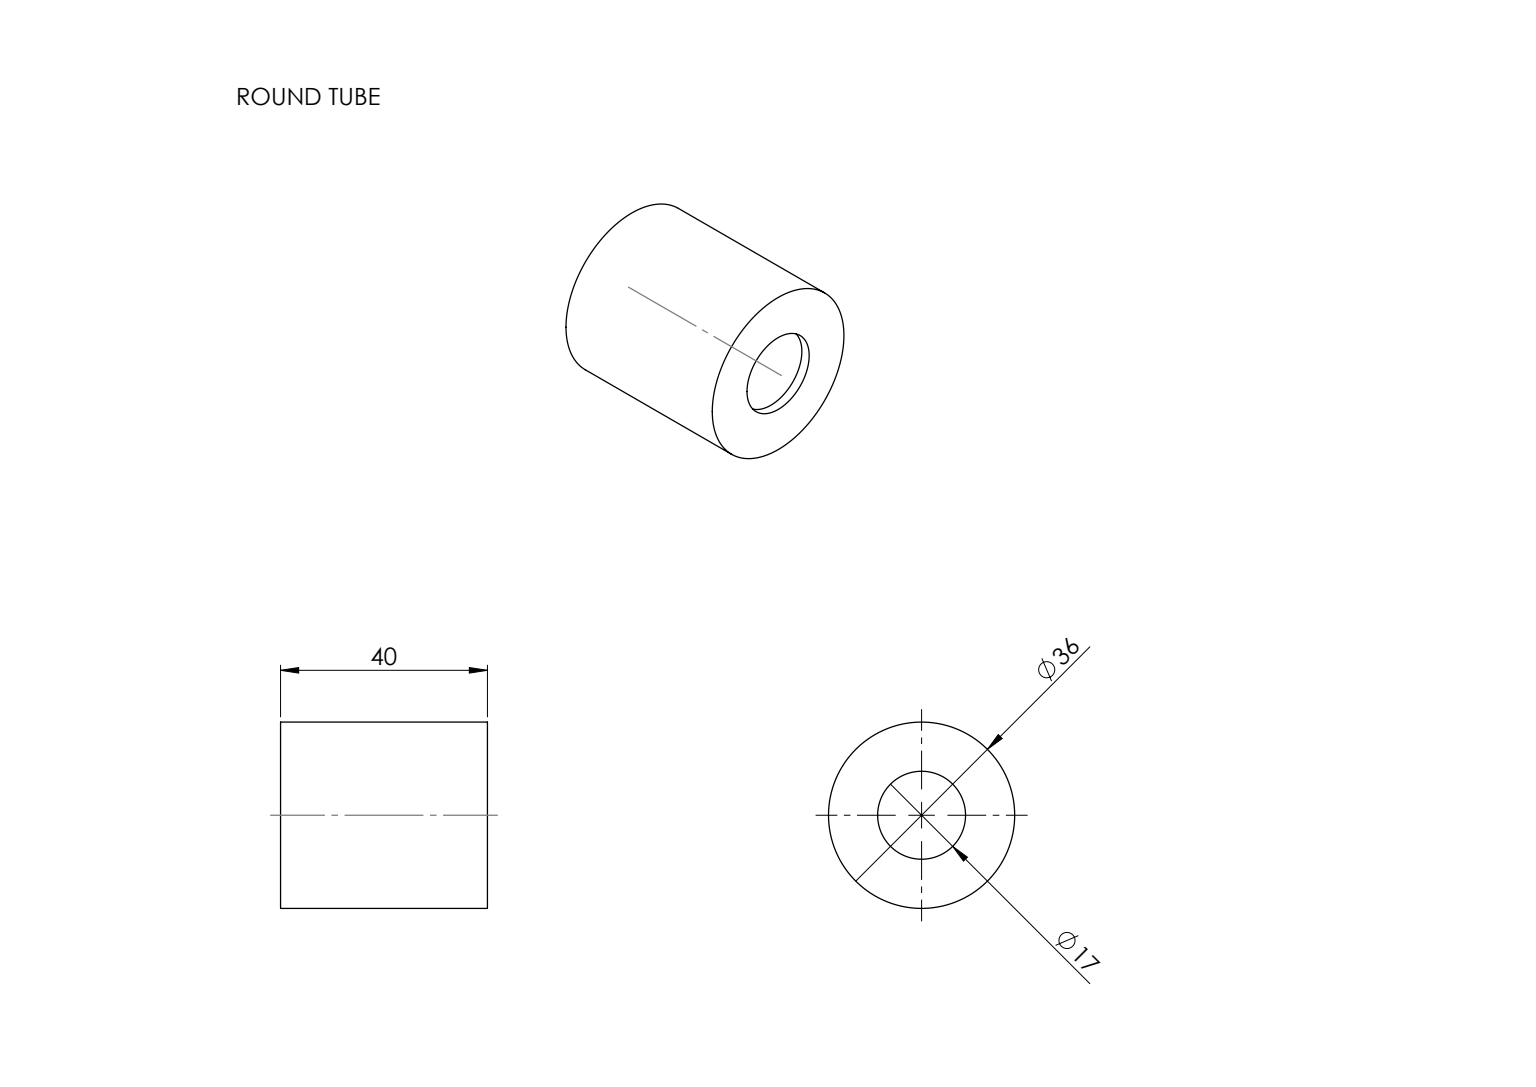
ISO-10303-21;
HEADER;
FILE_DESCRIPTION (('STEP AP214'),
    '1' );
FILE_NAME ('round tube.step',
    '2026-10-08T13:22:57',
    ( '' ),
    ( '' ),
    'SwSTEP 2.0',
    'SolidWorks 2026',
    '' );
FILE_SCHEMA (( 'AUTOMOTIVE_DESIGN' ));
ENDSEC;

DATA;
#17=DIRECTION ( 'NONE',  ( 0.000000000000000000, 0.000000000000000000, 1.000000000000000000 ) ) ;
#49=DIRECTION ( 'NONE',  ( -1.000000000000000000, 0.000000000000000000, -0.000000000000000000 ) ) ;
#62=CARTESIAN_POINT ( 'NONE',  ( -108.0000000000000284, 0.000000000000000000, 18.00000000000000000 ) ) ;
#71=FACE_OUTER_BOUND ( 'NONE', #2223, .T. ) ;
#103=EDGE_LOOP ( 'NONE', ( #4875, #2005 ) ) ;
#211=ADVANCED_FACE ( 'NONE', ( #9553 ), #5041, .F. ) ;
#245=CARTESIAN_POINT ( 'NONE',  ( 0.000000000000000000, 0.000000000000000000, 0.000000000000000000 ) ) ;
#254=MANIFOLD_SOLID_BREP ( 'Revolve-Thin1', #5480 ) ;
#268=EDGE_CURVE ( 'NONE', #3156, #7778, #4308, .T. ) ;
#280=FACE_OUTER_BOUND ( 'NONE', #4887, .T. ) ;
#290=EDGE_CURVE ( 'NONE', #9194, #8643, #8941, .T. ) ;
#357=( GEOMETRIC_REPRESENTATION_CONTEXT ( 3 ) GLOBAL_UNCERTAINTY_ASSIGNED_CONTEXT ( ( #1022 ) ) GLOBAL_UNIT_ASSIGNED_CONTEXT ( ( #599, #1315, #9183 ) ) REPRESENTATION_CONTEXT ( 'NONE', 'WORKASPACE' ) );
#358=( GEOMETRIC_REPRESENTATION_CONTEXT ( 3 ) GLOBAL_UNCERTAINTY_ASSIGNED_CONTEXT ( ( #7416 ) ) GLOBAL_UNIT_ASSIGNED_CONTEXT ( ( #3591, #997, #9684 ) ) REPRESENTATION_CONTEXT ( 'NONE', 'WORKASPACE' ) );
#438=EDGE_LOOP ( 'NONE', ( #4414, #892, #4751, #3837 ) ) ;
#465=ORIENTED_EDGE ( 'NONE', *, *, #2286, .F. ) ;
#494=PRODUCT_DEFINITION_CONTEXT ( 'detailed design', #8367, 'design' ) ;
#512=PRODUCT_CONTEXT ( 'NONE', #7716, 'mechanical' ) ;
#515=ORIENTED_EDGE ( 'NONE', *, *, #5831, .F. ) ;
#561=ADVANCED_FACE ( 'NONE', ( #71, #5593 ), #1530, .F. ) ;
#599=( LENGTH_UNIT ( ) NAMED_UNIT ( * ) SI_UNIT ( .MILLI., .METRE. ) );
#605=FILL_AREA_STYLE ('',( #8456 ) ) ;
#729=CARTESIAN_POINT ( 'NONE',  ( -108.0000000000000284, 2.204364238465235822E-15, -18.00000000000000355 ) ) ;
#740=EDGE_CURVE ( 'NONE', #7778, #3156, #4627, .T. ) ;
#763=DIRECTION ( 'NONE',  ( 0.000000000000000000, 0.000000000000000000, 1.000000000000000000 ) ) ;
#826=AXIS2_PLACEMENT_3D ( 'NONE', #1580, #4054, #7874 ) ;
#832=AXIS2_PLACEMENT_3D ( 'NONE', #8024, #7249, #6413 ) ;
#851=COLOUR_RGB ( '', 0.40784314, 0.44705882, 0.49803922) ;
#892=ORIENTED_EDGE ( 'NONE', *, *, #7551, .T. ) ;
#909=DIRECTION ( 'NONE',  ( -1.000000000000000000, -0.000000000000000000, -0.000000000000000000 ) ) ;
#932=ADVANCED_FACE ( 'NONE', ( #8639, #3149 ), #7183, .T. ) ;
#997=( NAMED_UNIT ( * ) PLANE_ANGLE_UNIT ( ) SI_UNIT ( $, .RADIAN. ) );
#1022=UNCERTAINTY_MEASURE_WITH_UNIT (LENGTH_MEASURE( 1.000000000000000082E-05 ), #599, 'distance_accuracy_value', 'NONE');
#1046=CIRCLE ( 'NONE', #1889, 15.99999999999999645 ) ;
#1072=CARTESIAN_POINT ( 'NONE',  ( -108.0000000000000284, 0.000000000000000000, 0.000000000000000000 ) ) ;
#1082=CYLINDRICAL_SURFACE ( 'NONE', #9749, 18.00000000000000355 ) ;
#1084=ORIENTED_EDGE ( 'NONE', *, *, #1371, .T. ) ;
#1137=ORIENTED_EDGE ( 'NONE', *, *, #2286, .T. ) ;
#1152=CARTESIAN_POINT ( 'NONE',  ( -108.0000000000000284, 0.000000000000000000, 0.000000000000000000 ) ) ;
#1175=ADVANCED_FACE ( 'NONE', ( #2510 ), #3234, .T. ) ;
#1211=LINE ( 'NONE', #6933, #2321 ) ;
#1315=( NAMED_UNIT ( * ) PLANE_ANGLE_UNIT ( ) SI_UNIT ( $, .RADIAN. ) );
#1371=EDGE_CURVE ( 'NONE', #3156, #3923, #3906, .T. ) ;
#1433=( LENGTH_UNIT ( ) NAMED_UNIT ( * ) SI_UNIT ( .MILLI., .METRE. ) );
#1457=CARTESIAN_POINT ( 'NONE',  ( -108.0000000000000284, 15.99999999999999645, 0.000000000000000000 ) ) ;
#1476=ADVANCED_FACE ( 'NONE', ( #9765 ), #1082, .T. ) ;
#1500=CARTESIAN_POINT ( 'NONE',  ( -108.0000000000000284, 0.000000000000000000, 15.99999999999999645 ) ) ;
#1517=COLOUR_RGB ( '', 0.40784314, 0.44705882, 0.49803922) ;
#1529=DIRECTION ( 'NONE',  ( -1.000000000000000000, 0.000000000000000000, -0.000000000000000000 ) ) ;
#1530=PLANE ( 'NONE',  #826 ) ;
#1577=CARTESIAN_POINT ( 'NONE',  ( -70.00000000000001421, 0.000000000000000000, 0.000000000000000000 ) ) ;
#1580=CARTESIAN_POINT ( 'NONE',  ( -68.00000000000001421, 8.500000000000000000, 0.000000000000000000 ) ) ;
#1624=CARTESIAN_POINT ( 'NONE',  ( -108.0000000000000284, 0.000000000000000000, 0.000000000000000000 ) ) ;
#1627=DIRECTION ( 'NONE',  ( -0.000000000000000000, 0.000000000000000000, 1.000000000000000000 ) ) ;
#1642=UNCERTAINTY_MEASURE_WITH_UNIT (LENGTH_MEASURE( 1.000000000000000082E-05 ), #1433, 'distance_accuracy_value', 'NONE');
#1673=DIRECTION ( 'NONE',  ( -1.000000000000000000, -0.000000000000000000, -0.000000000000000000 ) ) ;
#1678=CARTESIAN_POINT ( 'NONE',  ( -70.00000000000001421, 0.000000000000000000, 16.00000000000000000 ) ) ;
#1695=CARTESIAN_POINT ( 'NONE',  ( -108.0000000000000284, 0.000000000000000000, 0.000000000000000000 ) ) ;
#1829=CYLINDRICAL_SURFACE ( 'NONE', #3463, 16.00000000000000000 ) ;
#1832=AXIS2_PLACEMENT_3D ( 'NONE', #1072, #7466, #8187 ) ;
#1874=PRODUCT ( 'round tube', 'round tube', '', ( #512 ) ) ;
#1889=AXIS2_PLACEMENT_3D ( 'NONE', #1152, #1926, #9840 ) ;
#1926=DIRECTION ( 'NONE',  ( -1.000000000000000000, -0.000000000000000000, -0.000000000000000000 ) ) ;
#1927=CIRCLE ( 'NONE', #8535, 8.500000000000000000 ) ;
#1974=DIRECTION ( 'NONE',  ( 0.000000000000000000, 0.000000000000000000, 1.000000000000000000 ) ) ;
#2003=VERTEX_POINT ( 'NONE', #3029 ) ;
#2005=ORIENTED_EDGE ( 'NONE', *, *, #5772, .T. ) ;
#2018=CARTESIAN_POINT ( 'NONE',  ( -108.0000000000000284, 2.204364238465235428E-15, -18.00000000000000000 ) ) ;
#2037=PRODUCT_DEFINITION_SHAPE ( 'NONE', 'NONE',  #4346 ) ;
#2045=( NAMED_UNIT ( * ) SI_UNIT ( $, .STERADIAN. ) SOLID_ANGLE_UNIT ( ) );
#2095=AXIS2_PLACEMENT_3D ( 'NONE', #4772, #6463, #6557 ) ;
#2131=DIRECTION ( 'NONE',  ( -1.000000000000000000, -0.000000000000000000, -0.000000000000000000 ) ) ;
#2223=EDGE_LOOP ( 'NONE', ( #7638, #5766 ) ) ;
#2224=LINE ( 'NONE', #729, #9042 ) ;
#2228=EDGE_CURVE ( 'NONE', #6421, #9282, #4166, .T. ) ;
#2243=ORIENTED_EDGE ( 'NONE', *, *, #5831, .T. ) ;
#2252=DIRECTION ( 'NONE',  ( 0.000000000000000000, 0.000000000000000000, 1.000000000000000000 ) ) ;
#2286=EDGE_CURVE ( 'NONE', #9360, #3923, #3473, .T. ) ;
#2321=VECTOR ( 'NONE', #8550, 1000.000000000000000 ) ;
#2344=ORIENTED_EDGE ( 'NONE', *, *, #3789, .T. ) ;
#2413=ADVANCED_BREP_SHAPE_REPRESENTATION ( '', ( #254, #3995 ), #6945 ) ;
#2510=FACE_OUTER_BOUND ( 'NONE', #6282, .T. ) ;
#2527=VECTOR ( 'NONE', #6510, 1000.000000000000000 ) ;
#2554=CARTESIAN_POINT ( 'NONE',  ( -108.0000000000000284, 0.000000000000000000, 0.000000000000000000 ) ) ;
#2576=EDGE_LOOP ( 'NONE', ( #7299, #6905, #10175, #9434 ) ) ;
#2657=CARTESIAN_POINT ( 'NONE',  ( -108.0000000000000284, 0.000000000000000000, 0.000000000000000000 ) ) ;
#2669=DIRECTION ( 'NONE',  ( 0.000000000000000000, 0.000000000000000000, 1.000000000000000000 ) ) ;
#2678=ORIENTED_EDGE ( 'NONE', *, *, #5440, .F. ) ;
#2699=EDGE_CURVE ( 'NONE', #5232, #8643, #1211, .T. ) ;
#2721=ORIENTED_EDGE ( 'NONE', *, *, #8828, .F. ) ;
#2805=CIRCLE ( 'NONE', #8595, 18.00000000000000000 ) ;
#2816=CIRCLE ( 'NONE', #4642, 18.00000000000000355 ) ;
#2882=ORIENTED_EDGE ( 'NONE', *, *, #5772, .F. ) ;
#2885=ADVANCED_FACE ( 'NONE', ( #7092 ), #7730, .F. ) ;
#2988=AXIS2_PLACEMENT_3D ( 'NONE', #4365, #5955, #6053 ) ;
#3026=SURFACE_STYLE_USAGE ( .BOTH. , #3753 ) ;
#3029=CARTESIAN_POINT ( 'NONE',  ( -68.00000000000001421, 2.204364238465235822E-15, -18.00000000000000355 ) ) ;
#3066=EDGE_CURVE ( 'NONE', #6680, #9282, #1927, .T. ) ;
#3072=CARTESIAN_POINT ( 'NONE',  ( -68.00000000000001421, 0.000000000000000000, 0.000000000000000000 ) ) ;
#3149=FACE_BOUND ( 'NONE', #4435, .T. ) ;
#3156=VERTEX_POINT ( 'NONE', #1678 ) ;
#3186=AXIS2_PLACEMENT_3D ( 'NONE', #8225, #2131, #1974 ) ;
#3234=CYLINDRICAL_SURFACE ( 'NONE', #7095, 18.00000000000000355 ) ;
#3245=CARTESIAN_POINT ( 'NONE',  ( -108.0000000000000284, 0.000000000000000000, 0.000000000000000000 ) ) ;
#3271=CARTESIAN_POINT ( 'NONE',  ( -68.00000000000001421, 0.000000000000000000, 18.00000000000000355 ) ) ;
#3292=EDGE_CURVE ( 'NONE', #9282, #6680, #10186, .T. ) ;
#3294=DIRECTION ( 'NONE',  ( -1.000000000000000000, -0.000000000000000000, -0.000000000000000000 ) ) ;
#3339=DIRECTION ( 'NONE',  ( -1.000000000000000000, -0.000000000000000000, -0.000000000000000000 ) ) ;
#3453=STYLED_ITEM ( 'NONE', ( #5194 ), #254 ) ;
#3462=VECTOR ( 'NONE', #8822, 1000.000000000000000 ) ;
#3463=AXIS2_PLACEMENT_3D ( 'NONE', #2554, #909, #7928 ) ;
#3473=CIRCLE ( 'NONE', #9920, 15.99999999999999645 ) ;
#3502=EDGE_LOOP ( 'NONE', ( #9090, #6134 ) ) ;
#3591=( LENGTH_UNIT ( ) NAMED_UNIT ( * ) SI_UNIT ( .MILLI., .METRE. ) );
#3650=ORIENTED_EDGE ( 'NONE', *, *, #8828, .T. ) ;
#3753=SURFACE_SIDE_STYLE ('',( #6946 ) ) ;
#3789=EDGE_CURVE ( 'NONE', #2003, #9194, #2224, .T. ) ;
#3800=FACE_BOUND ( 'NONE', #10074, .T. ) ;
#3837=ORIENTED_EDGE ( 'NONE', *, *, #290, .F. ) ;
#3901=PLANE ( 'NONE',  #10093 ) ;
#3906=LINE ( 'NONE', #4060, #3462 ) ;
#3923=VERTEX_POINT ( 'NONE', #1500 ) ;
#3995=AXIS2_PLACEMENT_3D ( 'NONE', #245, #8930, #7419 ) ;
#4054=DIRECTION ( 'NONE',  ( -1.000000000000000000, 0.000000000000000000, -0.000000000000000000 ) ) ;
#4060=CARTESIAN_POINT ( 'NONE',  ( -108.0000000000000284, 0.000000000000000000, 16.00000000000000000 ) ) ;
#4104=CARTESIAN_POINT ( 'NONE',  ( -108.0000000000000284, 0.000000000000000000, 8.500000000000000000 ) ) ;
#4114=CARTESIAN_POINT ( 'NONE',  ( -108.0000000000000284, 1.040949779275250140E-15, -8.500000000000000000 ) ) ;
#4137=AXIS2_PLACEMENT_3D ( 'NONE', #3072, #6216, #8452 ) ;
#4166=LINE ( 'NONE', #4114, #4962 ) ;
#4168=DIRECTION ( 'NONE',  ( 0.000000000000000000, 0.000000000000000000, 1.000000000000000000 ) ) ;
#4201=LINE ( 'NONE', #4104, #2527 ) ;
#4259=ORIENTED_EDGE ( 'NONE', *, *, #290, .T. ) ;
#4308=CIRCLE ( 'NONE', #7941, 16.00000000000000000 ) ;
#4346=PRODUCT_DEFINITION ( 'UNKNOWN', '', #9394, #494 ) ;
#4352=AXIS2_PLACEMENT_3D ( 'NONE', #6148, #7768, #7815 ) ;
#4365=CARTESIAN_POINT ( 'NONE',  ( -108.0000000000000284, 0.000000000000000000, 0.000000000000000000 ) ) ;
#4414=ORIENTED_EDGE ( 'NONE', *, *, #3789, .F. ) ;
#4435=EDGE_LOOP ( 'NONE', ( #515, #465 ) ) ;
#4461=ORIENTED_EDGE ( 'NONE', *, *, #2699, .F. ) ;
#4464=AXIS2_PLACEMENT_3D ( 'NONE', #4630, #6262, #2252 ) ;
#4467=VECTOR ( 'NONE', #1673, 1000.000000000000000 ) ;
#4485=ORIENTED_EDGE ( 'NONE', *, *, #3292, .T. ) ;
#4526=FILL_AREA_STYLE_COLOUR ( '', #851 ) ;
#4534=CIRCLE ( 'NONE', #4352, 8.500000000000000000 ) ;
#4550=SHAPE_REPRESENTATION ( 'round tube', ( #3995 ), #6945 ) ;
#4575=DIRECTION ( 'NONE',  ( 0.000000000000000000, 0.000000000000000000, 1.000000000000000000 ) ) ;
#4627=CIRCLE ( 'NONE', #832, 16.00000000000000000 ) ;
#4630=CARTESIAN_POINT ( 'NONE',  ( -108.0000000000000284, 0.000000000000000000, 0.000000000000000000 ) ) ;
#4642=AXIS2_PLACEMENT_3D ( 'NONE', #5903, #9135, #4168 ) ;
#4648=AXIS2_PLACEMENT_3D ( 'NONE', #1624, #4675, #17 ) ;
#4675=DIRECTION ( 'NONE',  ( -1.000000000000000000, -0.000000000000000000, -0.000000000000000000 ) ) ;
#4751=ORIENTED_EDGE ( 'NONE', *, *, #2699, .T. ) ;
#4772=CARTESIAN_POINT ( 'NONE',  ( -70.00000000000001421, 0.000000000000000000, 0.000000000000000000 ) ) ;
#4875=ORIENTED_EDGE ( 'NONE', *, *, #6005, .T. ) ;
#4887=EDGE_LOOP ( 'NONE', ( #8548, #9088, #1137, #10177 ) ) ;
#4962=VECTOR ( 'NONE', #3339, 1000.000000000000000 ) ;
#5041=CYLINDRICAL_SURFACE ( 'NONE', #1832, 8.500000000000000000 ) ;
#5130=CIRCLE ( 'NONE', #4137, 18.00000000000000355 ) ;
#5154=ADVANCED_FACE ( 'NONE', ( #5546, #3800 ), #3901, .T. ) ;
#5194=PRESENTATION_STYLE_ASSIGNMENT (( #7683 ) ) ;
#5232=VERTEX_POINT ( 'NONE', #3271 ) ;
#5237=DIRECTION ( 'NONE',  ( -1.000000000000000000, -0.000000000000000000, -0.000000000000000000 ) ) ;
#5440=EDGE_CURVE ( 'NONE', #10061, #6680, #4201, .T. ) ;
#5445=CARTESIAN_POINT ( 'NONE',  ( -70.00000000000001421, 8.500000000000000000, 0.000000000000000000 ) ) ;
#5449=CARTESIAN_POINT ( 'NONE',  ( -70.00000000000001421, 1.959434878635765131E-15, -16.00000000000000000 ) ) ;
#5480=CLOSED_SHELL ( 'NONE', ( #8027, #211, #1175, #1476, #561, #2885, #5154, #7882, #932 ) ) ;
#5546=FACE_OUTER_BOUND ( 'NONE', #3502, .T. ) ;
#5593=FACE_BOUND ( 'NONE', #103, .T. ) ;
#5683=CARTESIAN_POINT ( 'NONE',  ( -68.00000000000001421, 1.040949779275250140E-15, -8.500000000000000000 ) ) ;
#5766=ORIENTED_EDGE ( 'NONE', *, *, #7551, .F. ) ;
#5772=EDGE_CURVE ( 'NONE', #6421, #10061, #7971, .T. ) ;
#5831=EDGE_CURVE ( 'NONE', #3923, #9360, #1046, .T. ) ;
#5903=CARTESIAN_POINT ( 'NONE',  ( -68.00000000000001421, 0.000000000000000000, 0.000000000000000000 ) ) ;
#5955=DIRECTION ( 'NONE',  ( -1.000000000000000000, -0.000000000000000000, -0.000000000000000000 ) ) ;
#6005=EDGE_CURVE ( 'NONE', #10061, #6421, #4534, .T. ) ;
#6053=DIRECTION ( 'NONE',  ( 0.000000000000000000, 0.000000000000000000, 1.000000000000000000 ) ) ;
#6134=ORIENTED_EDGE ( 'NONE', *, *, #740, .T. ) ;
#6148=CARTESIAN_POINT ( 'NONE',  ( -68.00000000000001421, 0.000000000000000000, 0.000000000000000000 ) ) ;
#6158=DIRECTION ( 'NONE',  ( -1.000000000000000000, -0.000000000000000000, -0.000000000000000000 ) ) ;
#6168=PRESENTATION_STYLE_ASSIGNMENT (( #3026 ) ) ;
#6216=DIRECTION ( 'NONE',  ( -1.000000000000000000, -0.000000000000000000, -0.000000000000000000 ) ) ;
#6262=DIRECTION ( 'NONE',  ( -1.000000000000000000, -0.000000000000000000, -0.000000000000000000 ) ) ;
#6282=EDGE_LOOP ( 'NONE', ( #7580, #2344, #2721, #4461 ) ) ;
#6355=CARTESIAN_POINT ( 'NONE',  ( -108.0000000000000284, 1.959434878635765131E-15, -16.00000000000000000 ) ) ;
#6413=DIRECTION ( 'NONE',  ( 0.000000000000000000, 0.000000000000000000, 1.000000000000000000 ) ) ;
#6421=VERTEX_POINT ( 'NONE', #5683 ) ;
#6463=DIRECTION ( 'NONE',  ( -1.000000000000000000, -0.000000000000000000, -0.000000000000000000 ) ) ;
#6510=DIRECTION ( 'NONE',  ( -1.000000000000000000, -0.000000000000000000, -0.000000000000000000 ) ) ;
#6551=CARTESIAN_POINT ( 'NONE',  ( -70.00000000000001421, 1.040949779275250140E-15, -8.500000000000000000 ) ) ;
#6557=DIRECTION ( 'NONE',  ( 0.000000000000000000, 0.000000000000000000, 1.000000000000000000 ) ) ;
#6680=VERTEX_POINT ( 'NONE', #8366 ) ;
#6795=SHAPE_DEFINITION_REPRESENTATION ( #2037, #4550 ) ;
#6905=ORIENTED_EDGE ( 'NONE', *, *, #6005, .F. ) ;
#6933=CARTESIAN_POINT ( 'NONE',  ( -108.0000000000000284, 0.000000000000000000, 18.00000000000000355 ) ) ;
#6945=( GEOMETRIC_REPRESENTATION_CONTEXT ( 3 ) GLOBAL_UNCERTAINTY_ASSIGNED_CONTEXT ( ( #1642 ) ) GLOBAL_UNIT_ASSIGNED_CONTEXT ( ( #1433, #9343, #2045 ) ) REPRESENTATION_CONTEXT ( 'NONE', 'WORKASPACE' ) );
#6946=SURFACE_STYLE_FILL_AREA ( #605 ) ;
#7025=DIRECTION ( 'NONE',  ( -0.000000000000000000, 0.000000000000000000, 1.000000000000000000 ) ) ;
#7049=FACE_OUTER_BOUND ( 'NONE', #7278, .T. ) ;
#7075=CARTESIAN_POINT ( 'NONE',  ( -68.00000000000001421, 0.000000000000000000, 8.500000000000000000 ) ) ;
#7086=LINE ( 'NONE', #6355, #4467 ) ;
#7092=FACE_OUTER_BOUND ( 'NONE', #2576, .T. ) ;
#7095=AXIS2_PLACEMENT_3D ( 'NONE', #1695, #7213, #763 ) ;
#7144=DIRECTION ( 'NONE',  ( -1.000000000000000000, -0.000000000000000000, -0.000000000000000000 ) ) ;
#7179=EDGE_CURVE ( 'NONE', #5232, #2003, #2816, .T. ) ;
#7183=PLANE ( 'NONE',  #8415 ) ;
#7213=DIRECTION ( 'NONE',  ( -1.000000000000000000, -0.000000000000000000, -0.000000000000000000 ) ) ;
#7249=DIRECTION ( 'NONE',  ( -1.000000000000000000, -0.000000000000000000, -0.000000000000000000 ) ) ;
#7278=EDGE_LOOP ( 'NONE', ( #9525, #8525, #1084, #2243 ) ) ;
#7299=ORIENTED_EDGE ( 'NONE', *, *, #2228, .F. ) ;
#7347=SHAPE_REPRESENTATION_RELATIONSHIP ( 'NONE' , 'NONE' ,  #4550, #2413 ) ;
#7411=DIRECTION ( 'NONE',  ( 0.000000000000000000, 0.000000000000000000, 1.000000000000000000 ) ) ;
#7416=UNCERTAINTY_MEASURE_WITH_UNIT (LENGTH_MEASURE( 1.000000000000000082E-05 ), #3591, 'distance_accuracy_value', 'NONE');
#7419=DIRECTION ( 'NONE',  ( 1.000000000000000000, 0.000000000000000000, 0.000000000000000000 ) ) ;
#7445=MECHANICAL_DESIGN_GEOMETRIC_PRESENTATION_REPRESENTATION('',(#3453),#357);
#7466=DIRECTION ( 'NONE',  ( -1.000000000000000000, -0.000000000000000000, -0.000000000000000000 ) ) ;
#7518=SURFACE_STYLE_FILL_AREA ( #7625 ) ;
#7551=EDGE_CURVE ( 'NONE', #2003, #5232, #5130, .T. ) ;
#7580=ORIENTED_EDGE ( 'NONE', *, *, #7179, .T. ) ;
#7625=FILL_AREA_STYLE ('',( #4526 ) ) ;
#7638=ORIENTED_EDGE ( 'NONE', *, *, #7179, .F. ) ;
#7683=SURFACE_STYLE_USAGE ( .BOTH. , #9955 ) ;
#7716=APPLICATION_CONTEXT ( 'automotive_design' ) ;
#7730=CYLINDRICAL_SURFACE ( 'NONE', #4648, 8.500000000000000000 ) ;
#7753=EDGE_LOOP ( 'NONE', ( #2882, #7908, #4485, #2678 ) ) ;
#7768=DIRECTION ( 'NONE',  ( -1.000000000000000000, -0.000000000000000000, -0.000000000000000000 ) ) ;
#7778=VERTEX_POINT ( 'NONE', #5449 ) ;
#7792=STYLED_ITEM ( 'NONE', ( #6168 ), #2413 ) ;
#7815=DIRECTION ( 'NONE',  ( 0.000000000000000000, 0.000000000000000000, 1.000000000000000000 ) ) ;
#7874=DIRECTION ( 'NONE',  ( -0.000000000000000000, 0.000000000000000000, 1.000000000000000000 ) ) ;
#7882=ADVANCED_FACE ( 'NONE', ( #7049 ), #9342, .F. ) ;
#7908=ORIENTED_EDGE ( 'NONE', *, *, #2228, .T. ) ;
#7928=DIRECTION ( 'NONE',  ( 0.000000000000000000, 0.000000000000000000, 1.000000000000000000 ) ) ;
#7941=AXIS2_PLACEMENT_3D ( 'NONE', #8342, #5237, #9901 ) ;
#7971=CIRCLE ( 'NONE', #3186, 8.500000000000000000 ) ;
#8024=CARTESIAN_POINT ( 'NONE',  ( -70.00000000000001421, 0.000000000000000000, 0.000000000000000000 ) ) ;
#8027=ADVANCED_FACE ( 'NONE', ( #280 ), #1829, .F. ) ;
#8068=DIRECTION ( 'NONE',  ( 0.000000000000000000, 0.000000000000000000, 1.000000000000000000 ) ) ;
#8135=DIRECTION ( 'NONE',  ( -1.000000000000000000, -0.000000000000000000, -0.000000000000000000 ) ) ;
#8187=DIRECTION ( 'NONE',  ( 0.000000000000000000, 0.000000000000000000, 1.000000000000000000 ) ) ;
#8197=ORIENTED_EDGE ( 'NONE', *, *, #3066, .F. ) ;
#8225=CARTESIAN_POINT ( 'NONE',  ( -68.00000000000001421, 0.000000000000000000, 0.000000000000000000 ) ) ;
#8342=CARTESIAN_POINT ( 'NONE',  ( -70.00000000000001421, 0.000000000000000000, 0.000000000000000000 ) ) ;
#8366=CARTESIAN_POINT ( 'NONE',  ( -70.00000000000001421, 0.000000000000000000, 8.500000000000000000 ) ) ;
#8367=APPLICATION_CONTEXT ( 'automotive_design' ) ;
#8415=AXIS2_PLACEMENT_3D ( 'NONE', #1457, #49, #7025 ) ;
#8452=DIRECTION ( 'NONE',  ( 0.000000000000000000, 0.000000000000000000, 1.000000000000000000 ) ) ;
#8456=FILL_AREA_STYLE_COLOUR ( '', #1517 ) ;
#8525=ORIENTED_EDGE ( 'NONE', *, *, #268, .F. ) ;
#8535=AXIS2_PLACEMENT_3D ( 'NONE', #1577, #6158, #4575 ) ;
#8548=ORIENTED_EDGE ( 'NONE', *, *, #740, .F. ) ;
#8550=DIRECTION ( 'NONE',  ( -1.000000000000000000, -0.000000000000000000, -0.000000000000000000 ) ) ;
#8595=AXIS2_PLACEMENT_3D ( 'NONE', #9581, #7144, #8068 ) ;
#8614=MECHANICAL_DESIGN_GEOMETRIC_PRESENTATION_REPRESENTATION('',(#7792),#358);
#8639=FACE_OUTER_BOUND ( 'NONE', #9147, .T. ) ;
#8643=VERTEX_POINT ( 'NONE', #62 ) ;
#8822=DIRECTION ( 'NONE',  ( -1.000000000000000000, -0.000000000000000000, -0.000000000000000000 ) ) ;
#8828=EDGE_CURVE ( 'NONE', #8643, #9194, #2805, .T. ) ;
#8842=EDGE_CURVE ( 'NONE', #7778, #9360, #7086, .T. ) ;
#8885=ORIENTED_EDGE ( 'NONE', *, *, #3292, .F. ) ;
#8930=DIRECTION ( 'NONE',  ( 0.000000000000000000, 0.000000000000000000, 1.000000000000000000 ) ) ;
#8941=CIRCLE ( 'NONE', #2988, 18.00000000000000000 ) ;
#9042=VECTOR ( 'NONE', #10127, 1000.000000000000000 ) ;
#9088=ORIENTED_EDGE ( 'NONE', *, *, #8842, .T. ) ;
#9090=ORIENTED_EDGE ( 'NONE', *, *, #268, .T. ) ;
#9135=DIRECTION ( 'NONE',  ( -1.000000000000000000, -0.000000000000000000, -0.000000000000000000 ) ) ;
#9147=EDGE_LOOP ( 'NONE', ( #3650, #4259 ) ) ;
#9183=( NAMED_UNIT ( * ) SI_UNIT ( $, .STERADIAN. ) SOLID_ANGLE_UNIT ( ) );
#9194=VERTEX_POINT ( 'NONE', #2018 ) ;
#9282=VERTEX_POINT ( 'NONE', #6551 ) ;
#9342=CYLINDRICAL_SURFACE ( 'NONE', #4464, 16.00000000000000000 ) ;
#9343=( NAMED_UNIT ( * ) PLANE_ANGLE_UNIT ( ) SI_UNIT ( $, .RADIAN. ) );
#9360=VERTEX_POINT ( 'NONE', #9734 ) ;
#9394=PRODUCT_DEFINITION_FORMATION_WITH_SPECIFIED_SOURCE ( 'ANY', '', #1874, .NOT_KNOWN. ) ;
#9434=ORIENTED_EDGE ( 'NONE', *, *, #3066, .T. ) ;
#9525=ORIENTED_EDGE ( 'NONE', *, *, #8842, .F. ) ;
#9553=FACE_OUTER_BOUND ( 'NONE', #7753, .T. ) ;
#9581=CARTESIAN_POINT ( 'NONE',  ( -108.0000000000000284, 0.000000000000000000, 0.000000000000000000 ) ) ;
#9684=( NAMED_UNIT ( * ) SI_UNIT ( $, .STERADIAN. ) SOLID_ANGLE_UNIT ( ) );
#9734=CARTESIAN_POINT ( 'NONE',  ( -108.0000000000000284, 1.959434878635764737E-15, -15.99999999999999645 ) ) ;
#9749=AXIS2_PLACEMENT_3D ( 'NONE', #3245, #3294, #2669 ) ;
#9765=FACE_OUTER_BOUND ( 'NONE', #438, .T. ) ;
#9840=DIRECTION ( 'NONE',  ( 0.000000000000000000, 0.000000000000000000, 1.000000000000000000 ) ) ;
#9901=DIRECTION ( 'NONE',  ( 0.000000000000000000, 0.000000000000000000, 1.000000000000000000 ) ) ;
#9920=AXIS2_PLACEMENT_3D ( 'NONE', #2657, #8135, #7411 ) ;
#9955=SURFACE_SIDE_STYLE ('',( #7518 ) ) ;
#10061=VERTEX_POINT ( 'NONE', #7075 ) ;
#10074=EDGE_LOOP ( 'NONE', ( #8197, #8885 ) ) ;
#10093=AXIS2_PLACEMENT_3D ( 'NONE', #5445, #1529, #1627 ) ;
#10127=DIRECTION ( 'NONE',  ( -1.000000000000000000, -0.000000000000000000, -0.000000000000000000 ) ) ;
#10175=ORIENTED_EDGE ( 'NONE', *, *, #5440, .T. ) ;
#10177=ORIENTED_EDGE ( 'NONE', *, *, #1371, .F. ) ;
#10186=CIRCLE ( 'NONE', #2095, 8.500000000000000000 ) ;
ENDSEC;
END-ISO-10303-21;
